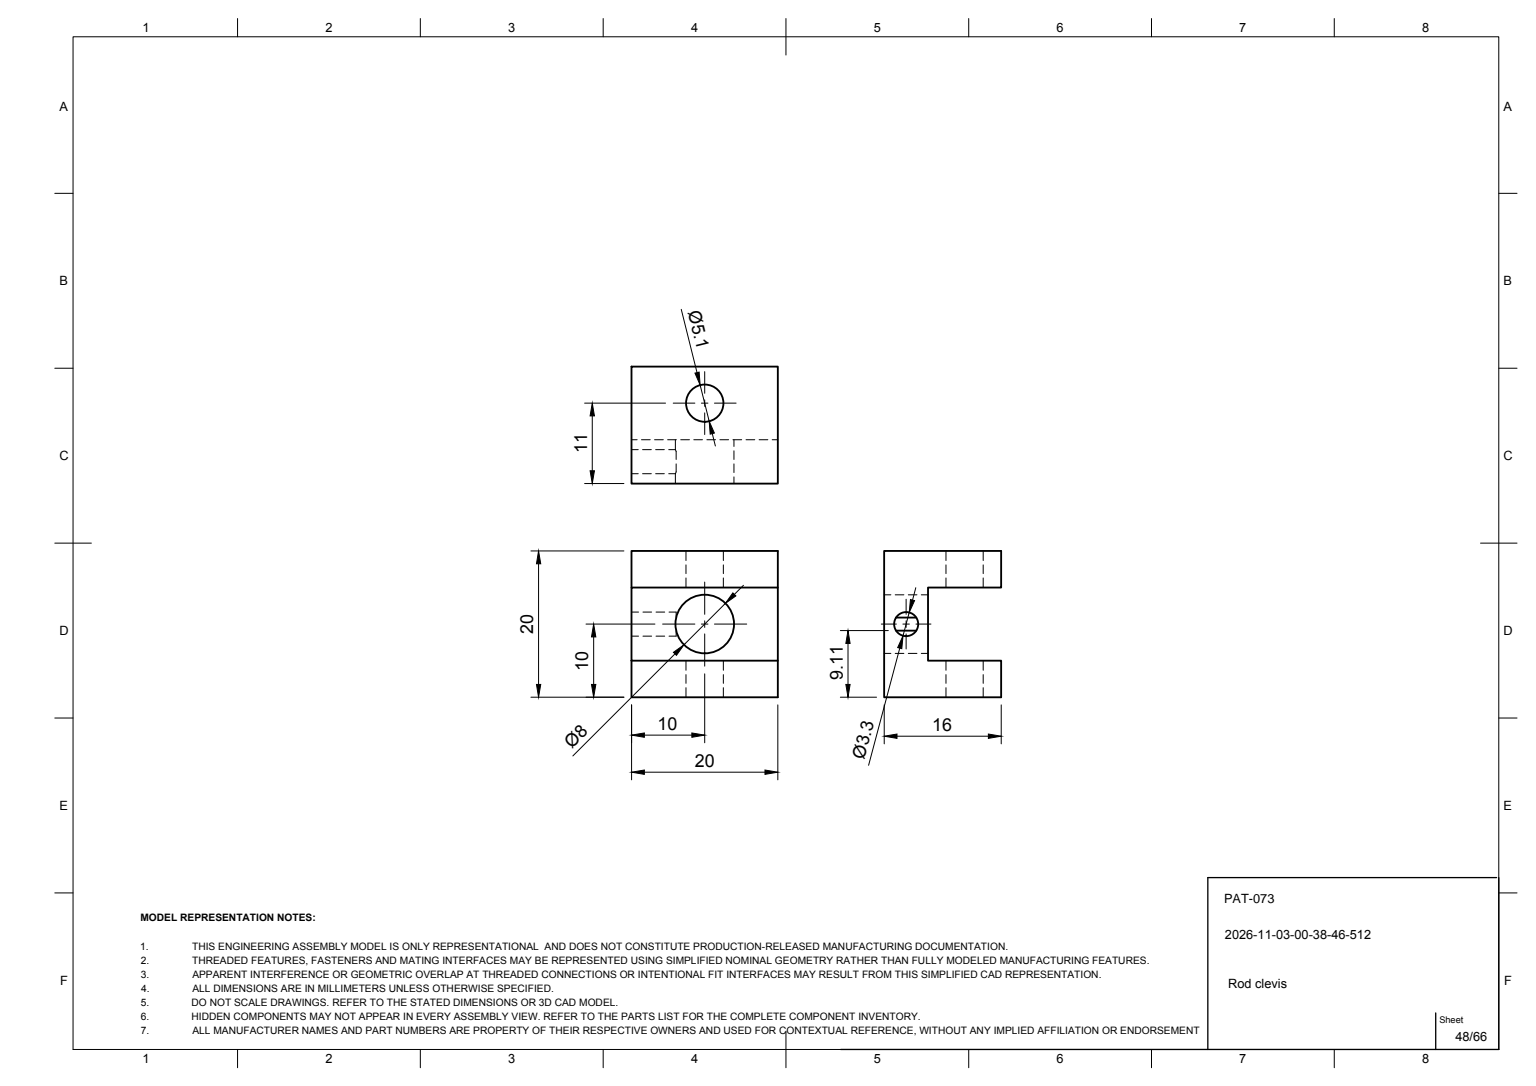
ISO-10303-21;
HEADER;
/* Generated by software containing ST-Developer
 * from STEP Tools, Inc. (www.steptools.com) 
 */

FILE_DESCRIPTION(
/* description */ ('Manual piston pump'),
/* implementation_level */ '2;1');

FILE_NAME(
/* name */ 'Rod clevis.step',
/* time_stamp */ '2026-11-02T16:54:23-08:00',
/* author */ (''),
/* organization */ (''),
/* preprocessor_version */ 'ST-DEVELOPER v20.2',
/* originating_system */ 'Autodesk Translation Framework v15.17.0.0',
/* authorisation */ '');

FILE_SCHEMA (('AUTOMOTIVE_DESIGN { 1 0 10303 214 3 1 1 }'));
ENDSEC;

DATA;
#10=MECHANICAL_DESIGN_GEOMETRIC_PRESENTATION_REPRESENTATION('',(#739),#19043);
#605=SHAPE_REPRESENTATION_RELATIONSHIP('SRR','None',#19354,#668);
#668=ADVANCED_BREP_SHAPE_REPRESENTATION('',(#808),#19021);
#739=STYLED_ITEM('',(#19661),#808);
#808=MANIFOLD_SOLID_BREP('Body1',#9526);
#1005=FACE_BOUND('',#2474,.T.);
#1006=FACE_BOUND('',#2476,.T.);
#1007=FACE_BOUND('',#2478,.T.);
#1008=FACE_BOUND('',#2480,.T.);
#1009=FACE_BOUND('',#2485,.T.);
#1010=FACE_BOUND('',#2487,.T.);
#1011=FACE_BOUND('',#2489,.T.);
#1012=FACE_BOUND('',#2491,.T.);
#1075=B_SPLINE_CURVE_WITH_KNOTS('',3,(#18004,#18005,#18006,#18007,#18008,
#18009,#18010,#18011,#18012,#18013),.UNSPECIFIED.,.F.,.F.,(4,2,2,2,4),(0.665271585430998,
0.692803751398643,0.75574615888762,0.818688566376597,0.846220732344242),
 .UNSPECIFIED.);
#1076=B_SPLINE_CURVE_WITH_KNOTS('',3,(#18021,#18022,#18023,#18024,#18025,
#18026,#18027,#18028,#18029,#18030),.UNSPECIFIED.,.F.,.F.,(4,2,2,2,4),(0.161440812839251,
0.188972978806896,0.251915386295873,0.31485779378485,0.342389959752495),
 .UNSPECIFIED.);
#1243=CYLINDRICAL_SURFACE('',#11104,0.165);
#1244=CYLINDRICAL_SURFACE('',#11109,0.255);
#1245=CYLINDRICAL_SURFACE('',#11112,0.255);
#1246=CYLINDRICAL_SURFACE('',#11115,0.4);
#1715=FACE_OUTER_BOUND('',#2468,.T.);
#1716=FACE_OUTER_BOUND('',#2469,.T.);
#1717=FACE_OUTER_BOUND('',#2470,.T.);
#1718=FACE_OUTER_BOUND('',#2471,.T.);
#1719=FACE_OUTER_BOUND('',#2472,.T.);
#1720=FACE_OUTER_BOUND('',#2473,.T.);
#1721=FACE_OUTER_BOUND('',#2475,.T.);
#1722=FACE_OUTER_BOUND('',#2477,.T.);
#1723=FACE_OUTER_BOUND('',#2479,.T.);
#1724=FACE_OUTER_BOUND('',#2481,.T.);
#1725=FACE_OUTER_BOUND('',#2482,.T.);
#1726=FACE_OUTER_BOUND('',#2483,.T.);
#1727=FACE_OUTER_BOUND('',#2484,.T.);
#1728=FACE_OUTER_BOUND('',#2486,.T.);
#1729=FACE_OUTER_BOUND('',#2488,.T.);
#1730=FACE_OUTER_BOUND('',#2490,.T.);
#2468=EDGE_LOOP('',(#7977,#7978));
#2469=EDGE_LOOP('',(#7979,#7980,#7981,#7982,#7983,#7984,#7985,#7986));
#2470=EDGE_LOOP('',(#7987,#7988,#7989));
#2471=EDGE_LOOP('',(#7990,#7991,#7992,#7993));
#2472=EDGE_LOOP('',(#7994,#7995,#7996,#7997));
#2473=EDGE_LOOP('',(#7998,#7999,#8000,#8001));
#2474=EDGE_LOOP('',(#8002,#8003,#8004,#8005));
#2475=EDGE_LOOP('',(#8006,#8007,#8008,#8009));
#2476=EDGE_LOOP('',(#8010));
#2477=EDGE_LOOP('',(#8011,#8012,#8013,#8014));
#2478=EDGE_LOOP('',(#8015));
#2479=EDGE_LOOP('',(#8016,#8017,#8018,#8019));
#2480=EDGE_LOOP('',(#8020));
#2481=EDGE_LOOP('',(#8021,#8022,#8023,#8024,#8025,#8026,#8027,#8028));
#2482=EDGE_LOOP('',(#8029,#8030,#8031,#8032));
#2483=EDGE_LOOP('',(#8033,#8034,#8035,#8036));
#2484=EDGE_LOOP('',(#8037,#8038,#8039,#8040));
#2485=EDGE_LOOP('',(#8041));
#2486=EDGE_LOOP('',(#8042,#8043,#8044,#8045));
#2487=EDGE_LOOP('',(#8046));
#2488=EDGE_LOOP('',(#8047,#8048,#8049,#8050));
#2489=EDGE_LOOP('',(#8051));
#2490=EDGE_LOOP('',(#8052,#8053,#8054,#8055,#8056,#8057,#8058,#8059));
#2491=EDGE_LOOP('',(#8060));
#3038=CIRCLE('',#11103,0.165);
#3039=CIRCLE('',#11105,0.165);
#3040=CIRCLE('',#11106,0.165);
#3041=CIRCLE('',#11107,0.165);
#3042=CIRCLE('',#11110,0.255);
#3043=CIRCLE('',#11111,0.255);
#3044=CIRCLE('',#11113,0.255);
#3045=CIRCLE('',#11114,0.255);
#3046=CIRCLE('',#11116,0.4);
#3047=CIRCLE('',#11117,0.4);
#3578=LINE('',#18000,#4182);
#3579=LINE('',#18017,#4183);
#3580=LINE('',#18032,#4184);
#3581=LINE('',#18037,#4185);
#3582=LINE('',#18043,#4186);
#3583=LINE('',#18049,#4187);
#3584=LINE('',#18054,#4188);
#3585=LINE('',#18056,#4189);
#3586=LINE('',#18058,#4190);
#3587=LINE('',#18059,#4191);
#3588=LINE('',#18062,#4192);
#3589=LINE('',#18064,#4193);
#3590=LINE('',#18065,#4194);
#3591=LINE('',#18068,#4195);
#3592=LINE('',#18070,#4196);
#3593=LINE('',#18071,#4197);
#3594=LINE('',#18074,#4198);
#3595=LINE('',#18076,#4199);
#3596=LINE('',#18078,#4200);
#3597=LINE('',#18080,#4201);
#3598=LINE('',#18081,#4202);
#3599=LINE('',#18084,#4203);
#3600=LINE('',#18085,#4204);
#3601=LINE('',#18088,#4205);
#3602=LINE('',#18089,#4206);
#3603=LINE('',#18092,#4207);
#3604=LINE('',#18094,#4208);
#3605=LINE('',#18095,#4209);
#3606=LINE('',#18097,#4210);
#3607=LINE('',#18099,#4211);
#4182=VECTOR('',#13646,1.);
#4183=VECTOR('',#13653,0.165);
#4184=VECTOR('',#13660,1.);
#4185=VECTOR('',#13665,0.255);
#4186=VECTOR('',#13672,0.255);
#4187=VECTOR('',#13679,0.4);
#4188=VECTOR('',#13684,1.);
#4189=VECTOR('',#13685,1.);
#4190=VECTOR('',#13686,1.);
#4191=VECTOR('',#13687,1.);
#4192=VECTOR('',#13690,1.);
#4193=VECTOR('',#13691,1.);
#4194=VECTOR('',#13692,1.);
#4195=VECTOR('',#13695,1.);
#4196=VECTOR('',#13696,1.);
#4197=VECTOR('',#13697,1.);
#4198=VECTOR('',#13700,1.);
#4199=VECTOR('',#13701,1.);
#4200=VECTOR('',#13702,1.);
#4201=VECTOR('',#13703,1.);
#4202=VECTOR('',#13704,1.);
#4203=VECTOR('',#13707,1.);
#4204=VECTOR('',#13708,1.);
#4205=VECTOR('',#13711,1.);
#4206=VECTOR('',#13712,1.);
#4207=VECTOR('',#13715,1.);
#4208=VECTOR('',#13716,1.);
#4209=VECTOR('',#13717,1.);
#4210=VECTOR('',#13720,1.);
#4211=VECTOR('',#13723,1.);
#4928=VERTEX_POINT('',#17998);
#4929=VERTEX_POINT('',#17999);
#4930=VERTEX_POINT('',#18003);
#4931=VERTEX_POINT('',#18014);
#4932=VERTEX_POINT('',#18016);
#4933=VERTEX_POINT('',#18019);
#4934=VERTEX_POINT('',#18034);
#4935=VERTEX_POINT('',#18036);
#4936=VERTEX_POINT('',#18040);
#4937=VERTEX_POINT('',#18042);
#4938=VERTEX_POINT('',#18046);
#4939=VERTEX_POINT('',#18048);
#4940=VERTEX_POINT('',#18052);
#4941=VERTEX_POINT('',#18053);
#4942=VERTEX_POINT('',#18055);
#4943=VERTEX_POINT('',#18057);
#4944=VERTEX_POINT('',#18061);
#4945=VERTEX_POINT('',#18063);
#4946=VERTEX_POINT('',#18067);
#4947=VERTEX_POINT('',#18069);
#4948=VERTEX_POINT('',#18073);
#4949=VERTEX_POINT('',#18075);
#4950=VERTEX_POINT('',#18077);
#4951=VERTEX_POINT('',#18079);
#4952=VERTEX_POINT('',#18083);
#4953=VERTEX_POINT('',#18087);
#4954=VERTEX_POINT('',#18091);
#4955=VERTEX_POINT('',#18093);
#5975=EDGE_CURVE('',#4928,#4929,#3578,.T.);
#5976=EDGE_CURVE('',#4928,#4929,#3038,.T.);
#5977=EDGE_CURVE('',#4930,#4928,#1075,.T.);
#5978=EDGE_CURVE('',#4931,#4930,#3039,.T.);
#5979=EDGE_CURVE('',#4931,#4932,#3579,.T.);
#5980=EDGE_CURVE('',#4932,#4932,#3040,.T.);
#5981=EDGE_CURVE('',#4933,#4931,#3041,.T.);
#5982=EDGE_CURVE('',#4929,#4933,#1076,.T.);
#5983=EDGE_CURVE('',#4933,#4930,#3580,.T.);
#5984=EDGE_CURVE('',#4934,#4934,#3042,.T.);
#5985=EDGE_CURVE('',#4934,#4935,#3581,.T.);
#5986=EDGE_CURVE('',#4935,#4935,#3043,.T.);
#5987=EDGE_CURVE('',#4936,#4936,#3044,.T.);
#5988=EDGE_CURVE('',#4936,#4937,#3582,.T.);
#5989=EDGE_CURVE('',#4937,#4937,#3045,.T.);
#5990=EDGE_CURVE('',#4938,#4938,#3046,.T.);
#5991=EDGE_CURVE('',#4938,#4939,#3583,.T.);
#5992=EDGE_CURVE('',#4939,#4939,#3047,.T.);
#5993=EDGE_CURVE('',#4940,#4941,#3584,.T.);
#5994=EDGE_CURVE('',#4942,#4940,#3585,.T.);
#5995=EDGE_CURVE('',#4943,#4942,#3586,.T.);
#5996=EDGE_CURVE('',#4941,#4943,#3587,.T.);
#5997=EDGE_CURVE('',#4944,#4940,#3588,.T.);
#5998=EDGE_CURVE('',#4945,#4944,#3589,.T.);
#5999=EDGE_CURVE('',#4942,#4945,#3590,.T.);
#6000=EDGE_CURVE('',#4946,#4944,#3591,.T.);
#6001=EDGE_CURVE('',#4947,#4946,#3592,.T.);
#6002=EDGE_CURVE('',#4945,#4947,#3593,.T.);
#6003=EDGE_CURVE('',#4948,#4947,#3594,.T.);
#6004=EDGE_CURVE('',#4949,#4948,#3595,.T.);
#6005=EDGE_CURVE('',#4950,#4949,#3596,.T.);
#6006=EDGE_CURVE('',#4951,#4950,#3597,.T.);
#6007=EDGE_CURVE('',#4943,#4951,#3598,.T.);
#6008=EDGE_CURVE('',#4952,#4946,#3599,.T.);
#6009=EDGE_CURVE('',#4948,#4952,#3600,.T.);
#6010=EDGE_CURVE('',#4951,#4953,#3601,.T.);
#6011=EDGE_CURVE('',#4941,#4953,#3602,.T.);
#6012=EDGE_CURVE('',#4949,#4954,#3603,.T.);
#6013=EDGE_CURVE('',#4955,#4954,#3604,.T.);
#6014=EDGE_CURVE('',#4950,#4955,#3605,.T.);
#6015=EDGE_CURVE('',#4953,#4955,#3606,.T.);
#6016=EDGE_CURVE('',#4954,#4952,#3607,.T.);
#7977=ORIENTED_EDGE('',*,*,#5975,.F.);
#7978=ORIENTED_EDGE('',*,*,#5976,.T.);
#7979=ORIENTED_EDGE('',*,*,#5977,.F.);
#7980=ORIENTED_EDGE('',*,*,#5978,.F.);
#7981=ORIENTED_EDGE('',*,*,#5979,.T.);
#7982=ORIENTED_EDGE('',*,*,#5980,.F.);
#7983=ORIENTED_EDGE('',*,*,#5979,.F.);
#7984=ORIENTED_EDGE('',*,*,#5981,.F.);
#7985=ORIENTED_EDGE('',*,*,#5982,.F.);
#7986=ORIENTED_EDGE('',*,*,#5976,.F.);
#7987=ORIENTED_EDGE('',*,*,#5983,.F.);
#7988=ORIENTED_EDGE('',*,*,#5981,.T.);
#7989=ORIENTED_EDGE('',*,*,#5978,.T.);
#7990=ORIENTED_EDGE('',*,*,#5984,.F.);
#7991=ORIENTED_EDGE('',*,*,#5985,.T.);
#7992=ORIENTED_EDGE('',*,*,#5986,.F.);
#7993=ORIENTED_EDGE('',*,*,#5985,.F.);
#7994=ORIENTED_EDGE('',*,*,#5987,.F.);
#7995=ORIENTED_EDGE('',*,*,#5988,.T.);
#7996=ORIENTED_EDGE('',*,*,#5989,.F.);
#7997=ORIENTED_EDGE('',*,*,#5988,.F.);
#7998=ORIENTED_EDGE('',*,*,#5990,.F.);
#7999=ORIENTED_EDGE('',*,*,#5991,.T.);
#8000=ORIENTED_EDGE('',*,*,#5992,.F.);
#8001=ORIENTED_EDGE('',*,*,#5991,.F.);
#8002=ORIENTED_EDGE('',*,*,#5982,.T.);
#8003=ORIENTED_EDGE('',*,*,#5983,.T.);
#8004=ORIENTED_EDGE('',*,*,#5977,.T.);
#8005=ORIENTED_EDGE('',*,*,#5975,.T.);
#8006=ORIENTED_EDGE('',*,*,#5993,.F.);
#8007=ORIENTED_EDGE('',*,*,#5994,.F.);
#8008=ORIENTED_EDGE('',*,*,#5995,.F.);
#8009=ORIENTED_EDGE('',*,*,#5996,.F.);
#8010=ORIENTED_EDGE('',*,*,#5987,.T.);
#8011=ORIENTED_EDGE('',*,*,#5997,.F.);
#8012=ORIENTED_EDGE('',*,*,#5998,.F.);
#8013=ORIENTED_EDGE('',*,*,#5999,.F.);
#8014=ORIENTED_EDGE('',*,*,#5994,.T.);
#8015=ORIENTED_EDGE('',*,*,#5990,.T.);
#8016=ORIENTED_EDGE('',*,*,#6000,.F.);
#8017=ORIENTED_EDGE('',*,*,#6001,.F.);
#8018=ORIENTED_EDGE('',*,*,#6002,.F.);
#8019=ORIENTED_EDGE('',*,*,#5998,.T.);
#8020=ORIENTED_EDGE('',*,*,#5986,.T.);
#8021=ORIENTED_EDGE('',*,*,#5995,.T.);
#8022=ORIENTED_EDGE('',*,*,#5999,.T.);
#8023=ORIENTED_EDGE('',*,*,#6002,.T.);
#8024=ORIENTED_EDGE('',*,*,#6003,.F.);
#8025=ORIENTED_EDGE('',*,*,#6004,.F.);
#8026=ORIENTED_EDGE('',*,*,#6005,.F.);
#8027=ORIENTED_EDGE('',*,*,#6006,.F.);
#8028=ORIENTED_EDGE('',*,*,#6007,.F.);
#8029=ORIENTED_EDGE('',*,*,#6001,.T.);
#8030=ORIENTED_EDGE('',*,*,#6008,.F.);
#8031=ORIENTED_EDGE('',*,*,#6009,.F.);
#8032=ORIENTED_EDGE('',*,*,#6003,.T.);
#8033=ORIENTED_EDGE('',*,*,#5996,.T.);
#8034=ORIENTED_EDGE('',*,*,#6007,.T.);
#8035=ORIENTED_EDGE('',*,*,#6010,.T.);
#8036=ORIENTED_EDGE('',*,*,#6011,.F.);
#8037=ORIENTED_EDGE('',*,*,#6005,.T.);
#8038=ORIENTED_EDGE('',*,*,#6012,.T.);
#8039=ORIENTED_EDGE('',*,*,#6013,.F.);
#8040=ORIENTED_EDGE('',*,*,#6014,.F.);
#8041=ORIENTED_EDGE('',*,*,#5992,.T.);
#8042=ORIENTED_EDGE('',*,*,#6006,.T.);
#8043=ORIENTED_EDGE('',*,*,#6014,.T.);
#8044=ORIENTED_EDGE('',*,*,#6015,.F.);
#8045=ORIENTED_EDGE('',*,*,#6010,.F.);
#8046=ORIENTED_EDGE('',*,*,#5989,.T.);
#8047=ORIENTED_EDGE('',*,*,#6004,.T.);
#8048=ORIENTED_EDGE('',*,*,#6009,.T.);
#8049=ORIENTED_EDGE('',*,*,#6016,.F.);
#8050=ORIENTED_EDGE('',*,*,#6012,.F.);
#8051=ORIENTED_EDGE('',*,*,#5984,.T.);
#8052=ORIENTED_EDGE('',*,*,#5993,.T.);
#8053=ORIENTED_EDGE('',*,*,#6011,.T.);
#8054=ORIENTED_EDGE('',*,*,#6015,.T.);
#8055=ORIENTED_EDGE('',*,*,#6013,.T.);
#8056=ORIENTED_EDGE('',*,*,#6016,.T.);
#8057=ORIENTED_EDGE('',*,*,#6008,.T.);
#8058=ORIENTED_EDGE('',*,*,#6000,.T.);
#8059=ORIENTED_EDGE('',*,*,#5997,.T.);
#8060=ORIENTED_EDGE('',*,*,#5980,.T.);
#8803=PLANE('',#11102);
#8804=PLANE('',#11108);
#8805=PLANE('',#11118);
#8806=PLANE('',#11119);
#8807=PLANE('',#11120);
#8808=PLANE('',#11121);
#8809=PLANE('',#11122);
#8810=PLANE('',#11123);
#8811=PLANE('',#11124);
#8812=PLANE('',#11125);
#8813=PLANE('',#11126);
#8814=PLANE('',#11127);
#9320=ADVANCED_FACE('',(#1715),#8803,.T.);
#9321=ADVANCED_FACE('',(#1716),#1243,.F.);
#9322=ADVANCED_FACE('',(#1717),#8804,.T.);
#9323=ADVANCED_FACE('',(#1718),#1244,.F.);
#9324=ADVANCED_FACE('',(#1719),#1245,.F.);
#9325=ADVANCED_FACE('',(#1720,#1005),#1246,.F.);
#9326=ADVANCED_FACE('',(#1721,#1006),#8805,.F.);
#9327=ADVANCED_FACE('',(#1722,#1007),#8806,.F.);
#9328=ADVANCED_FACE('',(#1723,#1008),#8807,.F.);
#9329=ADVANCED_FACE('',(#1724),#8808,.F.);
#9330=ADVANCED_FACE('',(#1725),#8809,.T.);
#9331=ADVANCED_FACE('',(#1726),#8810,.T.);
#9332=ADVANCED_FACE('',(#1727,#1009),#8811,.T.);
#9333=ADVANCED_FACE('',(#1728,#1010),#8812,.T.);
#9334=ADVANCED_FACE('',(#1729,#1011),#8813,.T.);
#9335=ADVANCED_FACE('',(#1730,#1012),#8814,.T.);
#9526=CLOSED_SHELL('',(#9320,#9321,#9322,#9323,#9324,#9325,#9326,#9327,
#9328,#9329,#9330,#9331,#9332,#9333,#9334,#9335));
#11101=AXIS2_PLACEMENT_3D('',#17996,#13642,#13643);
#11102=AXIS2_PLACEMENT_3D('',#17997,#13644,#13645);
#11103=AXIS2_PLACEMENT_3D('',#18001,#13647,#13648);
#11104=AXIS2_PLACEMENT_3D('',#18002,#13649,#13650);
#11105=AXIS2_PLACEMENT_3D('',#18015,#13651,#13652);
#11106=AXIS2_PLACEMENT_3D('',#18018,#13654,#13655);
#11107=AXIS2_PLACEMENT_3D('',#18020,#13656,#13657);
#11108=AXIS2_PLACEMENT_3D('',#18031,#13658,#13659);
#11109=AXIS2_PLACEMENT_3D('',#18033,#13661,#13662);
#11110=AXIS2_PLACEMENT_3D('',#18035,#13663,#13664);
#11111=AXIS2_PLACEMENT_3D('',#18038,#13666,#13667);
#11112=AXIS2_PLACEMENT_3D('',#18039,#13668,#13669);
#11113=AXIS2_PLACEMENT_3D('',#18041,#13670,#13671);
#11114=AXIS2_PLACEMENT_3D('',#18044,#13673,#13674);
#11115=AXIS2_PLACEMENT_3D('',#18045,#13675,#13676);
#11116=AXIS2_PLACEMENT_3D('',#18047,#13677,#13678);
#11117=AXIS2_PLACEMENT_3D('',#18050,#13680,#13681);
#11118=AXIS2_PLACEMENT_3D('',#18051,#13682,#13683);
#11119=AXIS2_PLACEMENT_3D('',#18060,#13688,#13689);
#11120=AXIS2_PLACEMENT_3D('',#18066,#13693,#13694);
#11121=AXIS2_PLACEMENT_3D('',#18072,#13698,#13699);
#11122=AXIS2_PLACEMENT_3D('',#18082,#13705,#13706);
#11123=AXIS2_PLACEMENT_3D('',#18086,#13709,#13710);
#11124=AXIS2_PLACEMENT_3D('',#18090,#13713,#13714);
#11125=AXIS2_PLACEMENT_3D('',#18096,#13718,#13719);
#11126=AXIS2_PLACEMENT_3D('',#18098,#13721,#13722);
#11127=AXIS2_PLACEMENT_3D('',#18100,#13724,#13725);
#13642=DIRECTION('axis',(0.,0.,1.));
#13643=DIRECTION('refdir',(1.,0.,0.));
#13644=DIRECTION('center_axis',(0.,0.,1.));
#13645=DIRECTION('ref_axis',(1.,0.,0.));
#13646=DIRECTION('',(0.,1.,0.));
#13647=DIRECTION('center_axis',(0.,0.,1.));
#13648=DIRECTION('ref_axis',(1.,0.,0.));
#13649=DIRECTION('center_axis',(0.,0.,1.));
#13650=DIRECTION('ref_axis',(1.,0.,0.));
#13651=DIRECTION('center_axis',(0.,0.,1.));
#13652=DIRECTION('ref_axis',(1.,0.,0.));
#13653=DIRECTION('',(0.,0.,1.));
#13654=DIRECTION('center_axis',(0.,0.,-1.));
#13655=DIRECTION('ref_axis',(1.,0.,0.));
#13656=DIRECTION('center_axis',(0.,0.,1.));
#13657=DIRECTION('ref_axis',(1.,0.,0.));
#13658=DIRECTION('center_axis',(0.,0.,1.));
#13659=DIRECTION('ref_axis',(1.,0.,0.));
#13660=DIRECTION('',(0.,-1.,0.));
#13661=DIRECTION('center_axis',(1.,0.,0.));
#13662=DIRECTION('ref_axis',(0.,0.,-1.));
#13663=DIRECTION('center_axis',(1.,0.,0.));
#13664=DIRECTION('ref_axis',(0.,0.,-1.));
#13665=DIRECTION('',(1.,0.,0.));
#13666=DIRECTION('center_axis',(-1.,0.,0.));
#13667=DIRECTION('ref_axis',(0.,0.,-1.));
#13668=DIRECTION('center_axis',(1.,0.,0.));
#13669=DIRECTION('ref_axis',(0.,0.,-1.));
#13670=DIRECTION('center_axis',(1.,0.,0.));
#13671=DIRECTION('ref_axis',(0.,0.,-1.));
#13672=DIRECTION('',(1.,0.,0.));
#13673=DIRECTION('center_axis',(-1.,0.,0.));
#13674=DIRECTION('ref_axis',(0.,0.,-1.));
#13675=DIRECTION('center_axis',(0.,1.,0.));
#13676=DIRECTION('ref_axis',(1.,0.,0.));
#13677=DIRECTION('center_axis',(0.,1.,0.));
#13678=DIRECTION('ref_axis',(1.,0.,0.));
#13679=DIRECTION('',(0.,1.,0.));
#13680=DIRECTION('center_axis',(0.,-1.,0.));
#13681=DIRECTION('ref_axis',(1.,0.,0.));
#13682=DIRECTION('center_axis',(1.,0.,0.));
#13683=DIRECTION('ref_axis',(0.,1.,0.));
#13684=DIRECTION('',(0.,-1.,0.));
#13685=DIRECTION('',(0.,0.,1.));
#13686=DIRECTION('',(0.,1.,0.));
#13687=DIRECTION('',(0.,0.,-1.));
#13688=DIRECTION('center_axis',(0.,1.,0.));
#13689=DIRECTION('ref_axis',(-1.,0.,0.));
#13690=DIRECTION('',(1.,0.,0.));
#13691=DIRECTION('',(0.,0.,1.));
#13692=DIRECTION('',(-1.,0.,0.));
#13693=DIRECTION('center_axis',(-1.,0.,0.));
#13694=DIRECTION('ref_axis',(0.,-1.,0.));
#13695=DIRECTION('',(0.,1.,0.));
#13696=DIRECTION('',(0.,0.,1.));
#13697=DIRECTION('',(0.,-1.,0.));
#13698=DIRECTION('center_axis',(0.,0.,1.));
#13699=DIRECTION('ref_axis',(1.,0.,0.));
#13700=DIRECTION('',(1.,0.,0.));
#13701=DIRECTION('',(0.,-1.,0.));
#13702=DIRECTION('',(-1.,0.,0.));
#13703=DIRECTION('',(0.,1.,0.));
#13704=DIRECTION('',(1.,0.,0.));
#13705=DIRECTION('center_axis',(0.,-1.,0.));
#13706=DIRECTION('ref_axis',(1.,0.,0.));
#13707=DIRECTION('',(1.,0.,0.));
#13708=DIRECTION('',(0.,0.,1.));
#13709=DIRECTION('center_axis',(0.,-1.,0.));
#13710=DIRECTION('ref_axis',(1.,0.,0.));
#13711=DIRECTION('',(0.,0.,1.));
#13712=DIRECTION('',(1.,0.,0.));
#13713=DIRECTION('center_axis',(0.,1.,0.));
#13714=DIRECTION('ref_axis',(-1.,0.,0.));
#13715=DIRECTION('',(0.,0.,1.));
#13716=DIRECTION('',(-1.,0.,0.));
#13717=DIRECTION('',(0.,0.,1.));
#13718=DIRECTION('center_axis',(1.,0.,0.));
#13719=DIRECTION('ref_axis',(0.,1.,0.));
#13720=DIRECTION('',(0.,1.,0.));
#13721=DIRECTION('center_axis',(-1.,0.,0.));
#13722=DIRECTION('ref_axis',(0.,-1.,0.));
#13723=DIRECTION('',(0.,-1.,0.));
#13724=DIRECTION('center_axis',(0.,0.,1.));
#13725=DIRECTION('ref_axis',(1.,0.,0.));
#17996=CARTESIAN_POINT('',(0.,0.,0.));
#17997=CARTESIAN_POINT('Origin',(0.,-5.3,4.89));
#17998=CARTESIAN_POINT('',(0.0888819441731535,-5.43901438774458,4.89));
#17999=CARTESIAN_POINT('',(0.0888819441731535,-5.16098561225542,4.89));
#18000=CARTESIAN_POINT('',(0.0888819441731535,-5.6,4.89));
#18001=CARTESIAN_POINT('Origin',(0.,-5.3,4.89));
#18002=CARTESIAN_POINT('Origin',(0.,-5.3,4.89));
#18003=CARTESIAN_POINT('',(-0.0888819441731535,-5.43901438774458,4.89));
#18004=CARTESIAN_POINT('Ctrl Pts',(-0.0888819441731541,-5.43901438774458,
4.89));
#18005=CARTESIAN_POINT('Ctrl Pts',(-0.0808964434200148,-5.44412009546053,
4.89181991495419));
#18006=CARTESIAN_POINT('Ctrl Pts',(-0.0723643333023662,-5.44859639186021,
4.89350251788328));
#18007=CARTESIAN_POINT('Ctrl Pts',(-0.0431949313468613,-5.46075622416973,
4.89819171553211));
#18008=CARTESIAN_POINT('Ctrl Pts',(-0.0209808024963256,-5.465,4.9));
#18009=CARTESIAN_POINT('Ctrl Pts',(0.0209808024963256,-5.465,4.9));
#18010=CARTESIAN_POINT('Ctrl Pts',(0.0431949313468613,-5.46075622416973,
4.89819171553211));
#18011=CARTESIAN_POINT('Ctrl Pts',(0.0723643333023662,-5.44859639186021,
4.89350251788328));
#18012=CARTESIAN_POINT('Ctrl Pts',(0.0808964434200144,-5.44412009546053,
4.89181991495419));
#18013=CARTESIAN_POINT('Ctrl Pts',(0.0888819441731541,-5.43901438774458,
4.89));
#18014=CARTESIAN_POINT('',(-0.165,-5.3,4.89));
#18015=CARTESIAN_POINT('Origin',(0.,-5.3,4.89));
#18016=CARTESIAN_POINT('',(-0.165,-5.3,5.5));
#18017=CARTESIAN_POINT('',(-0.165,-5.3,4.89));
#18018=CARTESIAN_POINT('Origin',(0.,-5.3,5.5));
#18019=CARTESIAN_POINT('',(-0.0888819441731535,-5.16098561225542,4.89));
#18020=CARTESIAN_POINT('Origin',(0.,-5.3,4.89));
#18021=CARTESIAN_POINT('Ctrl Pts',(0.0888819441731536,-5.16098561225542,
4.89));
#18022=CARTESIAN_POINT('Ctrl Pts',(0.0808964434200141,-5.15587990453947,
4.89181991495419));
#18023=CARTESIAN_POINT('Ctrl Pts',(0.0723643333023662,-5.15140360813979,
4.89350251788328));
#18024=CARTESIAN_POINT('Ctrl Pts',(0.0431949313468613,-5.13924377583027,
4.89819171553211));
#18025=CARTESIAN_POINT('Ctrl Pts',(0.0209808024963256,-5.135,4.9));
#18026=CARTESIAN_POINT('Ctrl Pts',(-0.0209808024963256,-5.135,4.9));
#18027=CARTESIAN_POINT('Ctrl Pts',(-0.0431949313468613,-5.13924377583027,
4.89819171553211));
#18028=CARTESIAN_POINT('Ctrl Pts',(-0.0723643333023663,-5.15140360813979,
4.89350251788328));
#18029=CARTESIAN_POINT('Ctrl Pts',(-0.0808964434200144,-5.15587990453947,
4.89181991495419));
#18030=CARTESIAN_POINT('Ctrl Pts',(-0.0888819441731536,-5.16098561225542,
4.89));
#18031=CARTESIAN_POINT('Origin',(0.,-5.3,4.89));
#18032=CARTESIAN_POINT('',(-0.0888819441731535,-5.6,4.89));
#18033=CARTESIAN_POINT('Origin',(-1.1,-6.1,4.5));
#18034=CARTESIAN_POINT('',(-1.,-6.1,4.755));
#18035=CARTESIAN_POINT('Origin',(-1.,-6.1,4.5));
#18036=CARTESIAN_POINT('',(-0.5,-6.1,4.755));
#18037=CARTESIAN_POINT('',(-1.1,-6.1,4.755));
#18038=CARTESIAN_POINT('Origin',(-0.5,-6.1,4.5));
#18039=CARTESIAN_POINT('Origin',(-1.1,-6.1,4.5));
#18040=CARTESIAN_POINT('',(0.5,-6.1,4.755));
#18041=CARTESIAN_POINT('Origin',(0.5,-6.1,4.5));
#18042=CARTESIAN_POINT('',(1.,-6.1,4.755));
#18043=CARTESIAN_POINT('',(-1.1,-6.1,4.755));
#18044=CARTESIAN_POINT('Origin',(1.,-6.1,4.5));
#18045=CARTESIAN_POINT('Origin',(0.,-5.6,4.5));
#18046=CARTESIAN_POINT('',(-0.4,-5.6,4.5));
#18047=CARTESIAN_POINT('Origin',(0.,-5.6,4.5));
#18048=CARTESIAN_POINT('',(-0.4,-5.,4.5));
#18049=CARTESIAN_POINT('',(-0.4,-5.6,4.5));
#18050=CARTESIAN_POINT('Origin',(0.,-5.,4.5));
#18051=CARTESIAN_POINT('Origin',(0.5,-6.7,3.4));
#18052=CARTESIAN_POINT('',(0.5,-5.6,5.5));
#18053=CARTESIAN_POINT('',(0.5,-6.6,5.5));
#18054=CARTESIAN_POINT('',(0.5,-6.25,5.5));
#18055=CARTESIAN_POINT('',(0.5,-5.6,3.5));
#18056=CARTESIAN_POINT('',(0.5,-5.6,3.4));
#18057=CARTESIAN_POINT('',(0.5,-6.6,3.5));
#18058=CARTESIAN_POINT('',(0.5,-6.25,3.5));
#18059=CARTESIAN_POINT('',(0.5,-6.6,3.45));
#18060=CARTESIAN_POINT('Origin',(0.5,-5.6,3.4));
#18061=CARTESIAN_POINT('',(-0.5,-5.6,5.5));
#18062=CARTESIAN_POINT('',(0.25,-5.6,5.5));
#18063=CARTESIAN_POINT('',(-0.5,-5.6,3.5));
#18064=CARTESIAN_POINT('',(-0.5,-5.6,3.4));
#18065=CARTESIAN_POINT('',(0.25,-5.6,3.5));
#18066=CARTESIAN_POINT('Origin',(-0.5,-5.6,3.4));
#18067=CARTESIAN_POINT('',(-0.5,-6.6,5.5));
#18068=CARTESIAN_POINT('',(-0.5,-5.7,5.5));
#18069=CARTESIAN_POINT('',(-0.5,-6.6,3.5));
#18070=CARTESIAN_POINT('',(-0.5,-6.6,3.45));
#18071=CARTESIAN_POINT('',(-0.5,-5.7,3.5));
#18072=CARTESIAN_POINT('Origin',(0.,-5.8,3.5));
#18073=CARTESIAN_POINT('',(-1.,-6.6,3.5));
#18074=CARTESIAN_POINT('',(-1.,-6.6,3.5));
#18075=CARTESIAN_POINT('',(-1.,-5.,3.5));
#18076=CARTESIAN_POINT('',(-1.,-5.,3.5));
#18077=CARTESIAN_POINT('',(1.,-5.,3.5));
#18078=CARTESIAN_POINT('',(1.,-5.,3.5));
#18079=CARTESIAN_POINT('',(1.,-6.6,3.5));
#18080=CARTESIAN_POINT('',(1.,-6.6,3.5));
#18081=CARTESIAN_POINT('',(-1.,-6.6,3.5));
#18082=CARTESIAN_POINT('Origin',(-1.,-6.6,3.5));
#18083=CARTESIAN_POINT('',(-1.,-6.6,5.5));
#18084=CARTESIAN_POINT('',(-1.,-6.6,5.5));
#18085=CARTESIAN_POINT('',(-1.,-6.6,3.5));
#18086=CARTESIAN_POINT('Origin',(-1.,-6.6,3.5));
#18087=CARTESIAN_POINT('',(1.,-6.6,5.5));
#18088=CARTESIAN_POINT('',(1.,-6.6,3.5));
#18089=CARTESIAN_POINT('',(-1.,-6.6,5.5));
#18090=CARTESIAN_POINT('Origin',(1.,-5.,3.5));
#18091=CARTESIAN_POINT('',(-1.,-5.,5.5));
#18092=CARTESIAN_POINT('',(-1.,-5.,3.5));
#18093=CARTESIAN_POINT('',(1.,-5.,5.5));
#18094=CARTESIAN_POINT('',(1.,-5.,5.5));
#18095=CARTESIAN_POINT('',(1.,-5.,3.5));
#18096=CARTESIAN_POINT('Origin',(1.,-6.6,3.5));
#18097=CARTESIAN_POINT('',(1.,-6.6,5.5));
#18098=CARTESIAN_POINT('Origin',(-1.,-5.,3.5));
#18099=CARTESIAN_POINT('',(-1.,-5.,5.5));
#18100=CARTESIAN_POINT('Origin',(0.,-5.8,5.5));
#18950=UNCERTAINTY_MEASURE_WITH_UNIT(LENGTH_MEASURE(0.001),#19044,
'DISTANCE_ACCURACY_VALUE',
'Maximum model space distance between geometric entities at asserted c
onnectivities');
#18972=UNCERTAINTY_MEASURE_WITH_UNIT(LENGTH_MEASURE(0.001),#19044,
'DISTANCE_ACCURACY_VALUE',
'Maximum model space distance between geometric entities at asserted c
onnectivities');
#19021=(
GEOMETRIC_REPRESENTATION_CONTEXT(3)
GLOBAL_UNCERTAINTY_ASSIGNED_CONTEXT((#18950))
GLOBAL_UNIT_ASSIGNED_CONTEXT((#19044,#19046,#19047))
REPRESENTATION_CONTEXT('','3D')
);
#19043=(
GEOMETRIC_REPRESENTATION_CONTEXT(3)
GLOBAL_UNCERTAINTY_ASSIGNED_CONTEXT((#18972))
GLOBAL_UNIT_ASSIGNED_CONTEXT((#19044,#19046,#19047))
REPRESENTATION_CONTEXT('','3D')
);
#19044=(
LENGTH_UNIT()
NAMED_UNIT(*)
SI_UNIT(.CENTI.,.METRE.)
);
#19046=(
NAMED_UNIT(*)
PLANE_ANGLE_UNIT()
SI_UNIT($,.RADIAN.)
);
#19047=(
NAMED_UNIT(*)
SI_UNIT($,.STERADIAN.)
SOLID_ANGLE_UNIT()
);
#19096=SHAPE_DEFINITION_REPRESENTATION(#19173,#19354);
#19173=PRODUCT_DEFINITION_SHAPE('',$,#19425);
#19354=SHAPE_REPRESENTATION('',(#11101),#19021);
#19376=PRODUCT_DEFINITION_CONTEXT('part definition',#19588,'design');
#19425=PRODUCT_DEFINITION('2026-11-03-00-38-46-512','Rod clevis',#19495,
#19376);
#19495=PRODUCT_DEFINITION_FORMATION('',$,#19638);
#19588=APPLICATION_CONTEXT(
'Core Data for Automotive Mechanical Design Process');
#19589=PRODUCT_CONTEXT('part definition',#19588,'mechanical');
#19638=PRODUCT('2026-11-03-00-38-46-512','Rod clevis','Rod clevis',(#19589));
#19661=PRESENTATION_STYLE_ASSIGNMENT((#19667));
#19667=SURFACE_STYLE_USAGE(.BOTH.,#19673);
#19673=SURFACE_SIDE_STYLE('',(#19679));
#19679=SURFACE_STYLE_FILL_AREA(#19685);
#19685=FILL_AREA_STYLE('CAD Library Painted - Engineering blue',(#19691));
#19691=FILL_AREA_STYLE_COLOUR('CAD Library Painted - Engineering blue',
#19697);
#19697=COLOUR_RGB('CAD Library Painted - Engineering blue',0.12156862745098,
0.356862745098039,0.6);
ENDSEC;
END-ISO-10303-21;
